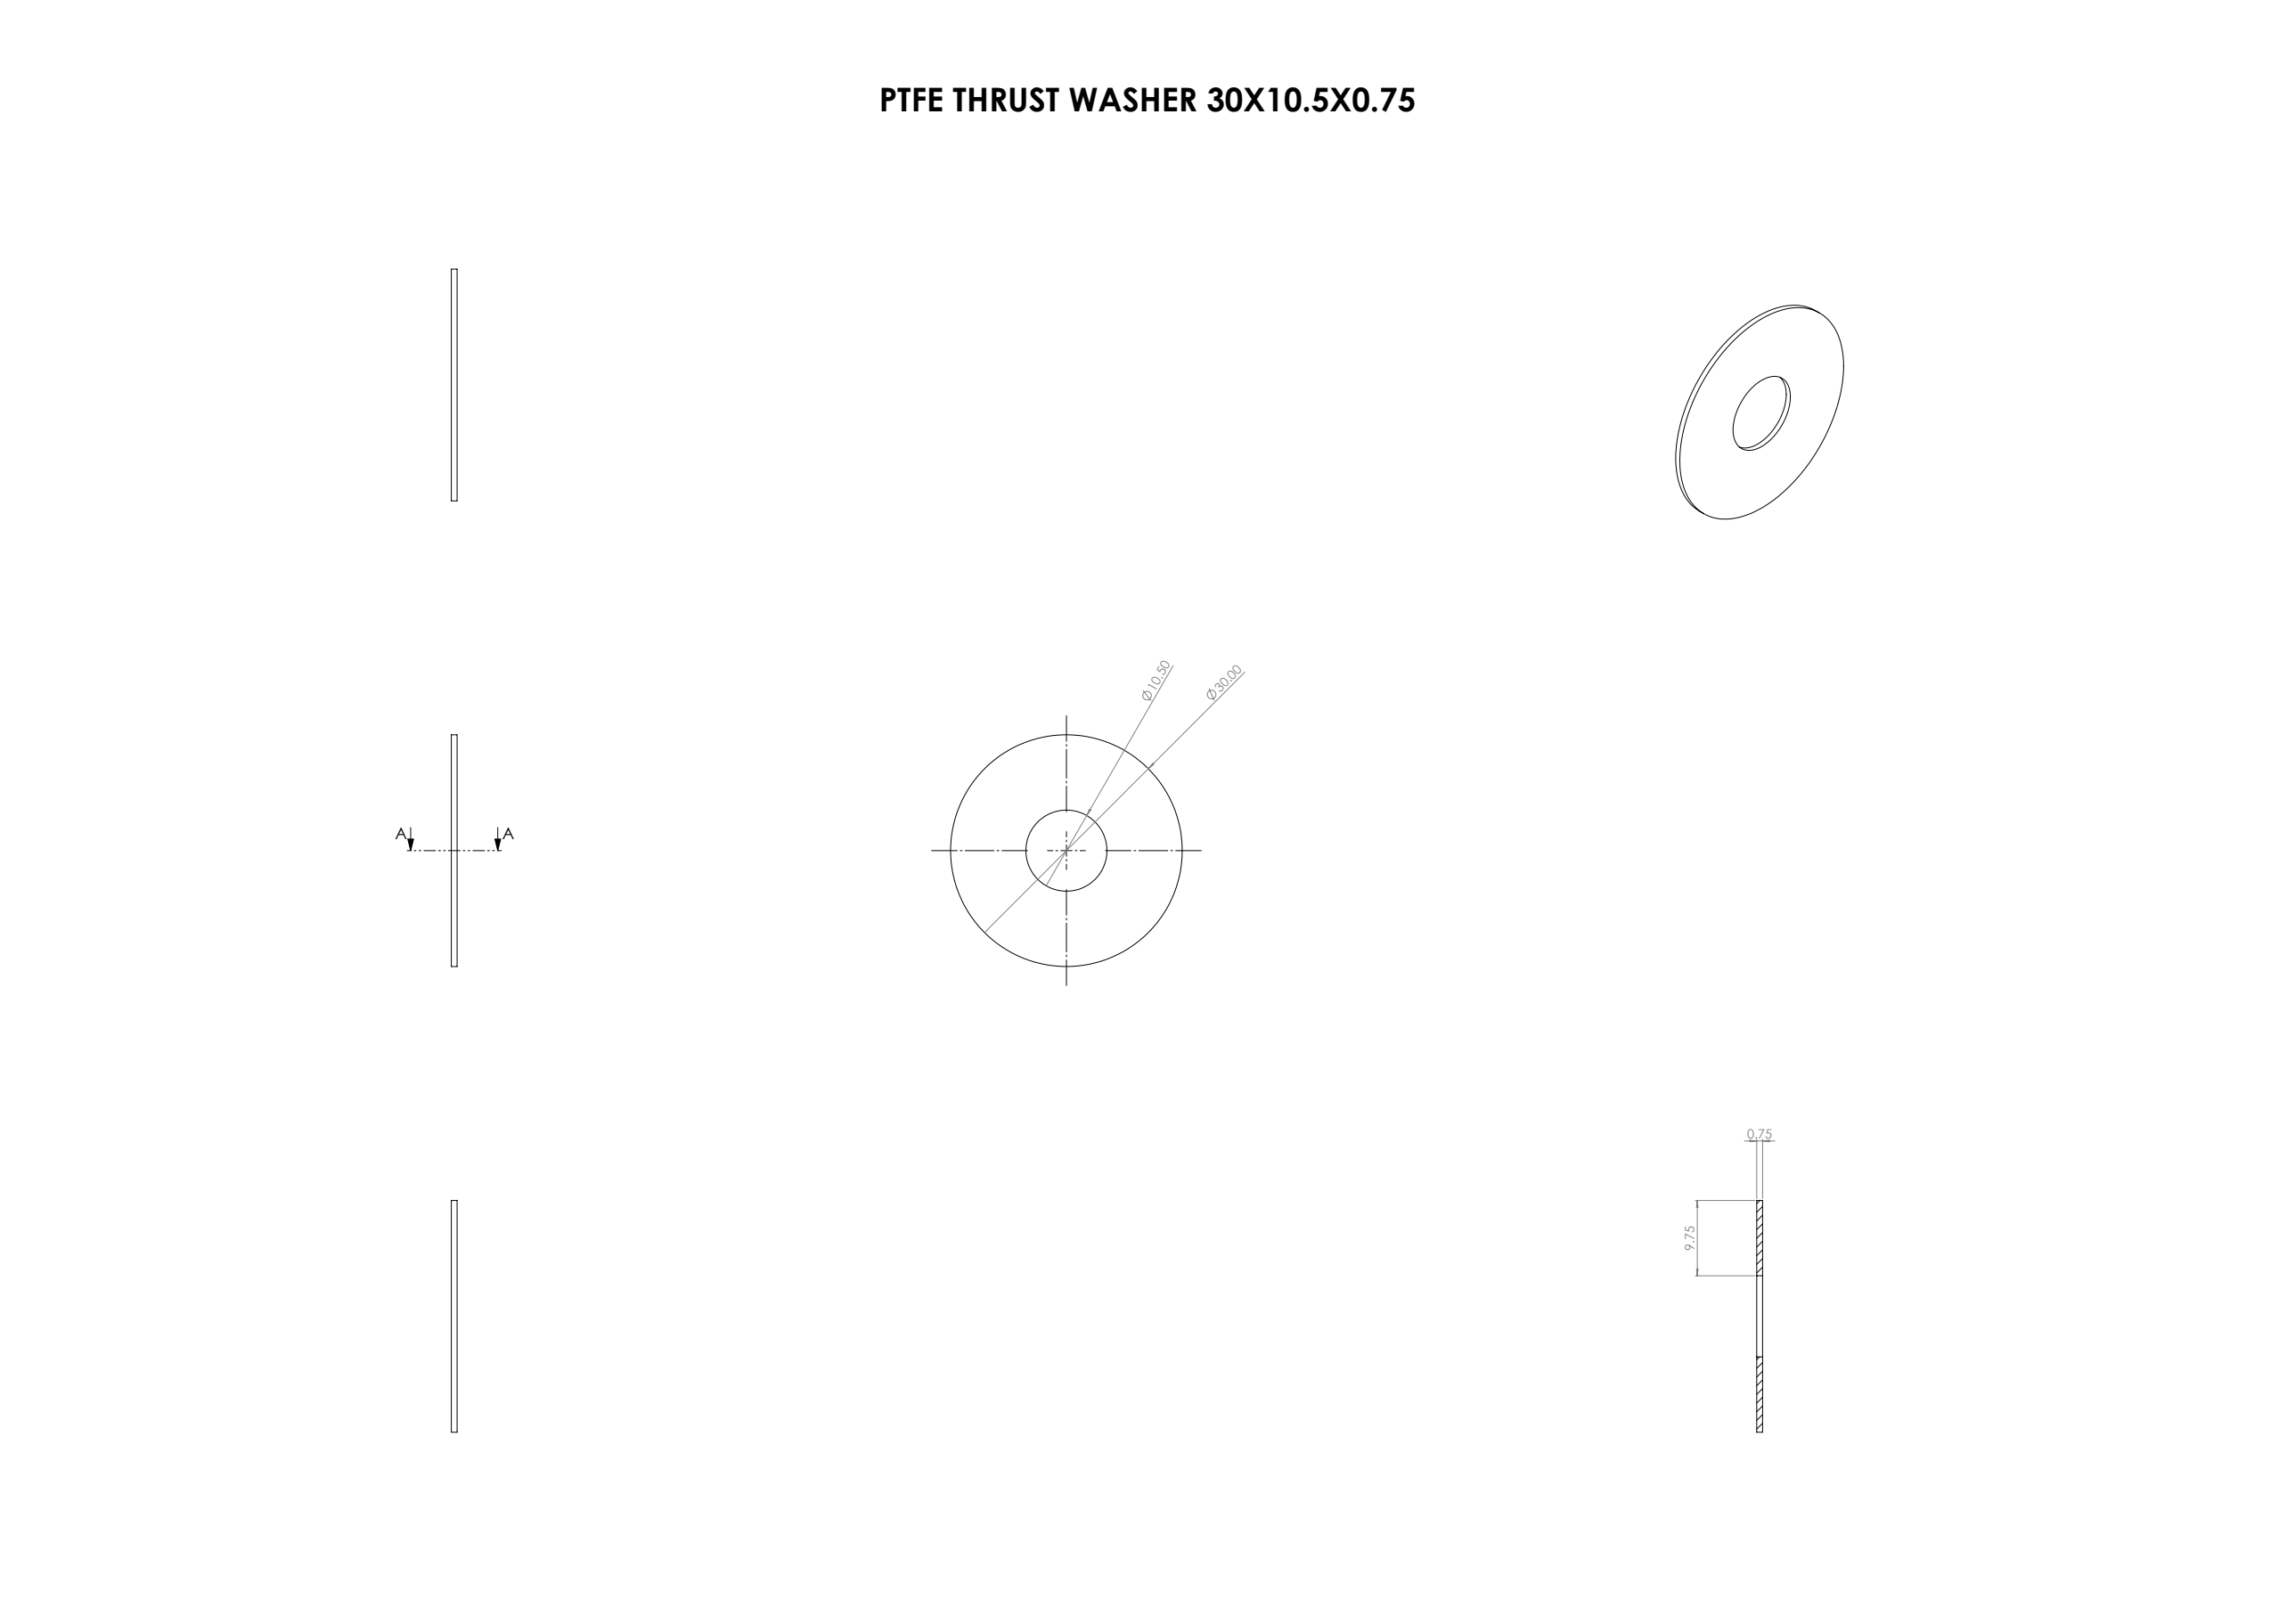
ISO-10303-21;
HEADER;
/* Generated by software containing ST-Developer
 * from STEP Tools, Inc. (www.steptools.com) 
 */

FILE_DESCRIPTION(
/* description */ (''),
/* implementation_level */ '2;1');

FILE_NAME(
/* name */ '12_PTFE_Thrust_Washer_30x10.5x0.75.step',
/* time_stamp */ '2026-10-21T01:56:51-07:00',
/* author */ (''),
/* organization */ (''),
/* preprocessor_version */ 'ST-DEVELOPER v20.2',
/* originating_system */ 'Autodesk Translation Framework v15.15.0.0',
/* authorisation */ '');

FILE_SCHEMA (('AUTOMOTIVE_DESIGN { 1 0 10303 214 3 1 1 }'));
ENDSEC;

DATA;
#10=MECHANICAL_DESIGN_GEOMETRIC_PRESENTATION_REPRESENTATION('',(#276),#82384);
#238=SHAPE_REPRESENTATION_RELATIONSHIP('SRR','None',#82472,#257);
#257=ADVANCED_BREP_SHAPE_REPRESENTATION('',(#295),#82371);
#276=STYLED_ITEM('',(#82638),#295);
#295=MANIFOLD_SOLID_BREP('Body1',#30667);
#573=CYLINDRICAL_SURFACE('',#32067,5.25);
#574=CYLINDRICAL_SURFACE('',#32072,15.);
#1524=CIRCLE('',#32068,5.25);
#1525=CIRCLE('',#32069,5.25);
#1526=CIRCLE('',#32071,15.);
#1527=CIRCLE('',#32073,15.);
#3484=FACE_BOUND('',#6329,.T.);
#3485=FACE_BOUND('',#6332,.T.);
#4371=FACE_OUTER_BOUND('',#6327,.T.);
#4372=FACE_OUTER_BOUND('',#6328,.T.);
#4373=FACE_OUTER_BOUND('',#6330,.T.);
#4374=FACE_OUTER_BOUND('',#6331,.T.);
#6327=EDGE_LOOP('',(#23027,#23028,#23029,#23030));
#6328=EDGE_LOOP('',(#23031));
#6329=EDGE_LOOP('',(#23032));
#6330=EDGE_LOOP('',(#23033,#23034,#23035,#23036));
#6331=EDGE_LOOP('',(#23037));
#6332=EDGE_LOOP('',(#23038));
#8474=LINE('',#48878,#10780);
#8475=LINE('',#48886,#10781);
#10780=VECTOR('',#36863,5.25);
#10781=VECTOR('',#36874,15.);
#13175=VERTEX_POINT('',#48875);
#13176=VERTEX_POINT('',#48877);
#13177=VERTEX_POINT('',#48881);
#13178=VERTEX_POINT('',#48884);
#16735=EDGE_CURVE('',#13175,#13175,#1524,.T.);
#16736=EDGE_CURVE('',#13175,#13176,#8474,.T.);
#16737=EDGE_CURVE('',#13176,#13176,#1525,.T.);
#16738=EDGE_CURVE('',#13177,#13177,#1526,.T.);
#16739=EDGE_CURVE('',#13178,#13178,#1527,.T.);
#16740=EDGE_CURVE('',#13178,#13177,#8475,.T.);
#23027=ORIENTED_EDGE('',*,*,#16735,.T.);
#23028=ORIENTED_EDGE('',*,*,#16736,.T.);
#23029=ORIENTED_EDGE('',*,*,#16737,.F.);
#23030=ORIENTED_EDGE('',*,*,#16736,.F.);
#23031=ORIENTED_EDGE('',*,*,#16738,.F.);
#23032=ORIENTED_EDGE('',*,*,#16737,.T.);
#23033=ORIENTED_EDGE('',*,*,#16739,.F.);
#23034=ORIENTED_EDGE('',*,*,#16740,.T.);
#23035=ORIENTED_EDGE('',*,*,#16738,.T.);
#23036=ORIENTED_EDGE('',*,*,#16740,.F.);
#23037=ORIENTED_EDGE('',*,*,#16739,.T.);
#23038=ORIENTED_EDGE('',*,*,#16735,.F.);
#28470=PLANE('',#32070);
#28471=PLANE('',#32074);
#29699=ADVANCED_FACE('',(#4371),#573,.F.);
#29700=ADVANCED_FACE('',(#4372,#3484),#28470,.T.);
#29701=ADVANCED_FACE('',(#4373),#574,.T.);
#29702=ADVANCED_FACE('',(#4374,#3485),#28471,.T.);
#30667=CLOSED_SHELL('',(#29699,#29700,#29701,#29702));
#32066=AXIS2_PLACEMENT_3D('',#48873,#36857,#36858);
#32067=AXIS2_PLACEMENT_3D('',#48874,#36859,#36860);
#32068=AXIS2_PLACEMENT_3D('',#48876,#36861,#36862);
#32069=AXIS2_PLACEMENT_3D('',#48879,#36864,#36865);
#32070=AXIS2_PLACEMENT_3D('',#48880,#36866,#36867);
#32071=AXIS2_PLACEMENT_3D('',#48882,#36868,#36869);
#32072=AXIS2_PLACEMENT_3D('',#48883,#36870,#36871);
#32073=AXIS2_PLACEMENT_3D('',#48885,#36872,#36873);
#32074=AXIS2_PLACEMENT_3D('',#48887,#36875,#36876);
#36857=DIRECTION('axis',(0.,0.,1.));
#36858=DIRECTION('refdir',(1.,0.,0.));
#36859=DIRECTION('center_axis',(1.,0.,0.));
#36860=DIRECTION('ref_axis',(0.,1.,0.));
#36861=DIRECTION('center_axis',(1.,0.,0.));
#36862=DIRECTION('ref_axis',(0.,0.,-1.));
#36863=DIRECTION('',(-1.,0.,0.));
#36864=DIRECTION('center_axis',(1.,0.,0.));
#36865=DIRECTION('ref_axis',(0.,0.,-1.));
#36866=DIRECTION('center_axis',(-1.,0.,0.));
#36867=DIRECTION('ref_axis',(0.,0.,1.));
#36868=DIRECTION('center_axis',(1.,0.,0.));
#36869=DIRECTION('ref_axis',(0.,0.,-1.));
#36870=DIRECTION('center_axis',(1.,0.,0.));
#36871=DIRECTION('ref_axis',(0.,1.,0.));
#36872=DIRECTION('center_axis',(1.,0.,0.));
#36873=DIRECTION('ref_axis',(0.,0.,-1.));
#36874=DIRECTION('',(-1.,0.,0.));
#36875=DIRECTION('center_axis',(1.,0.,0.));
#36876=DIRECTION('ref_axis',(0.,0.,-1.));
#48873=CARTESIAN_POINT('',(0.,0.,0.));
#48874=CARTESIAN_POINT('Origin',(0.375,0.,0.));
#48875=CARTESIAN_POINT('',(0.75,-5.25,-6.42939569552361E-16));
#48876=CARTESIAN_POINT('Origin',(0.75,0.,0.));
#48877=CARTESIAN_POINT('',(0.,-5.25,-6.42939569552361E-16));
#48878=CARTESIAN_POINT('',(0.375,-5.25,-6.42939569552361E-16));
#48879=CARTESIAN_POINT('Origin',(0.,0.,0.));
#48880=CARTESIAN_POINT('Origin',(0.,15.,0.));
#48881=CARTESIAN_POINT('',(0.,-15.,-1.83697019872103E-15));
#48882=CARTESIAN_POINT('Origin',(0.,0.,0.));
#48883=CARTESIAN_POINT('Origin',(0.375,0.,0.));
#48884=CARTESIAN_POINT('',(0.75,-15.,-1.83697019872103E-15));
#48885=CARTESIAN_POINT('Origin',(0.75,0.,0.));
#48886=CARTESIAN_POINT('',(0.375,-15.,-1.83697019872103E-15));
#48887=CARTESIAN_POINT('Origin',(0.75,5.25,0.));
#82350=UNCERTAINTY_MEASURE_WITH_UNIT(LENGTH_MEASURE(0.01),#82385,
'DISTANCE_ACCURACY_VALUE',
'Maximum model space distance between geometric entities at asserted c
onnectivities');
#82363=UNCERTAINTY_MEASURE_WITH_UNIT(LENGTH_MEASURE(0.01),#82385,
'DISTANCE_ACCURACY_VALUE',
'Maximum model space distance between geometric entities at asserted c
onnectivities');
#82371=(
GEOMETRIC_REPRESENTATION_CONTEXT(3)
GLOBAL_UNCERTAINTY_ASSIGNED_CONTEXT((#82350))
GLOBAL_UNIT_ASSIGNED_CONTEXT((#82385,#82387,#82388))
REPRESENTATION_CONTEXT('','3D')
);
#82384=(
GEOMETRIC_REPRESENTATION_CONTEXT(3)
GLOBAL_UNCERTAINTY_ASSIGNED_CONTEXT((#82363))
GLOBAL_UNIT_ASSIGNED_CONTEXT((#82385,#82387,#82388))
REPRESENTATION_CONTEXT('','3D')
);
#82385=(
LENGTH_UNIT()
NAMED_UNIT(*)
SI_UNIT(.MILLI.,.METRE.)
);
#82387=(
NAMED_UNIT(*)
PLANE_ANGLE_UNIT()
SI_UNIT($,.RADIAN.)
);
#82388=(
NAMED_UNIT(*)
SI_UNIT($,.STERADIAN.)
SOLID_ANGLE_UNIT()
);
#82396=SHAPE_DEFINITION_REPRESENTATION(#82416,#82472);
#82416=PRODUCT_DEFINITION_SHAPE('',$,#82493);
#82472=SHAPE_REPRESENTATION('',(#32066),#82371);
#82485=PRODUCT_DEFINITION_CONTEXT('part definition',#82547,'design');
#82493=PRODUCT_DEFINITION('2026-10-20-12-38-23-638',
'12_PTFE_Thrust_Washer_30x10.5x0.75',#82513,#82485);
#82513=PRODUCT_DEFINITION_FORMATION('',$,#82556);
#82547=APPLICATION_CONTEXT(
'Core Data for Automotive Mechanical Design Process');
#82548=PRODUCT_CONTEXT('part definition',#82547,'mechanical');
#82556=PRODUCT('2026-10-20-12-38-23-638',
'12_PTFE_Thrust_Washer_30x10.5x0.75',$,(#82548));
#82632=COLOUR_RGB('Black',0.12,0.14,0.17);
#82633=FILL_AREA_STYLE_COLOUR('',#82632);
#82634=FILL_AREA_STYLE('',(#82633));
#82635=SURFACE_STYLE_FILL_AREA(#82634);
#82636=SURFACE_SIDE_STYLE('',(#82635));
#82637=SURFACE_STYLE_USAGE(.BOTH.,#82636);
#82638=PRESENTATION_STYLE_ASSIGNMENT((#82637));
ENDSEC;
END-ISO-10303-21;
